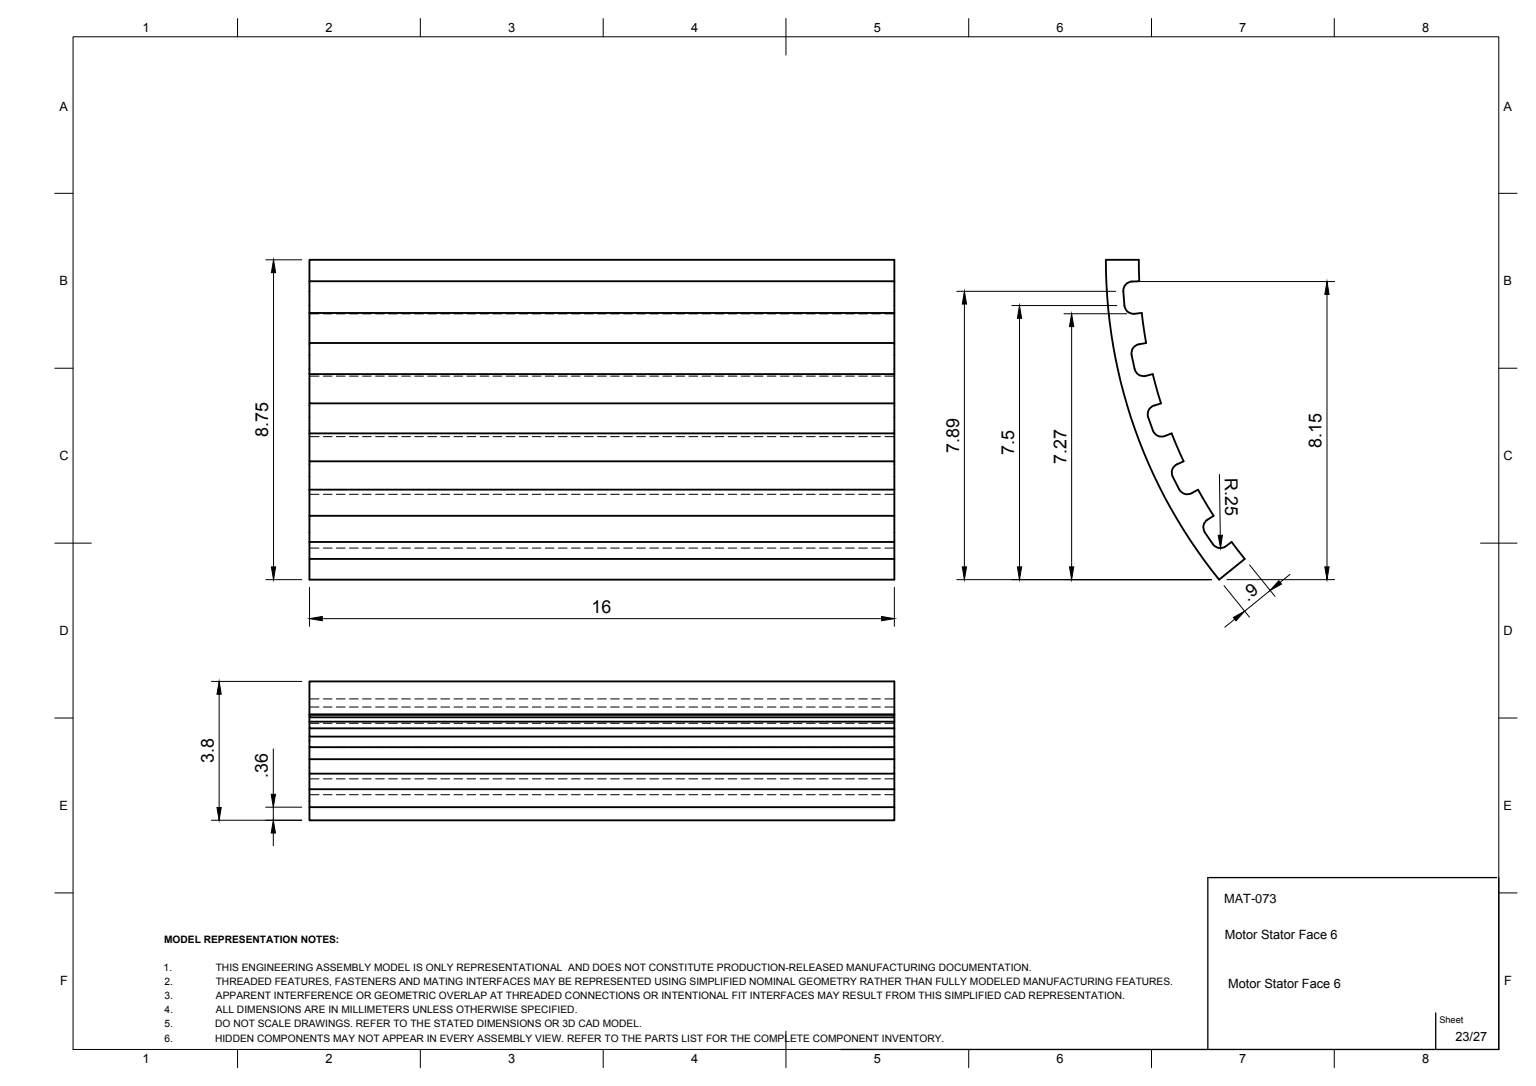
ISO-10303-21;
HEADER;
/* Generated by software containing ST-Developer
 * from STEP Tools, Inc. (www.steptools.com) 
 */

FILE_DESCRIPTION(
/* description */ ('CAx-IF Rec.Pracs.---Representation and Presentation of Product Manufa
cturing Information (PMI)---4.0---2014-10-13'),
/* implementation_level */ '2;1');

FILE_NAME(
/* name */ 'Motor Stator Face 6.step',
/* time_stamp */ '2026-10-24T18:52:33-07:00',
/* author */ (''),
/* organization */ (''),
/* preprocessor_version */ 'ST-DEVELOPER v20.2',
/* originating_system */ 'Autodesk Translation Framework v15.17.0.0',
/* authorisation */ '');

FILE_SCHEMA (('AP242_MANAGED_MODEL_BASED_3D_ENGINEERING_MIM_LF { 1 0 10303 442 2 1 4 }'));
ENDSEC;

DATA;
#10=MECHANICAL_DESIGN_GEOMETRIC_PRESENTATION_REPRESENTATION('',(#439),#34876);
#373=SHAPE_REPRESENTATION_RELATIONSHIP('SRR','None',#35010,#406);
#406=ADVANCED_BREP_SHAPE_REPRESENTATION('',(#472),#34868);
#439=STYLED_ITEM('',(#35160),#472);
#472=MANIFOLD_SOLID_BREP('Motor Stator Face 6',#19579);
#965=PLANE('',#21833);
#966=PLANE('',#21843);
#967=PLANE('',#21853);
#968=PLANE('',#21863);
#969=PLANE('',#21873);
#970=PLANE('',#21874);
#971=PLANE('',#21875);
#972=PLANE('',#21876);
#973=PLANE('',#21877);
#974=PLANE('',#21884);
#975=PLANE('',#21894);
#976=PLANE('',#21899);
#977=PLANE('',#21902);
#978=PLANE('',#21903);
#2305=LINE('',#33385,#3904);
#2306=LINE('',#33388,#3905);
#2307=LINE('',#33393,#3906);
#2308=LINE('',#33399,#3907);
#2309=LINE('',#33403,#3908);
#2310=LINE('',#33405,#3909);
#2311=LINE('',#33406,#3910);
#2312=LINE('',#33412,#3911);
#2313=LINE('',#33415,#3912);
#2314=LINE('',#33420,#3913);
#2315=LINE('',#33426,#3914);
#2316=LINE('',#33430,#3915);
#2317=LINE('',#33432,#3916);
#2318=LINE('',#33433,#3917);
#2319=LINE('',#33439,#3918);
#2320=LINE('',#33442,#3919);
#2321=LINE('',#33447,#3920);
#2322=LINE('',#33453,#3921);
#2323=LINE('',#33457,#3922);
#2324=LINE('',#33459,#3923);
#2325=LINE('',#33460,#3924);
#2326=LINE('',#33466,#3925);
#2327=LINE('',#33469,#3926);
#2328=LINE('',#33474,#3927);
#2329=LINE('',#33480,#3928);
#2330=LINE('',#33484,#3929);
#2331=LINE('',#33486,#3930);
#2332=LINE('',#33487,#3931);
#2333=LINE('',#33493,#3932);
#2334=LINE('',#33496,#3933);
#2335=LINE('',#33501,#3934);
#2336=LINE('',#33507,#3935);
#2337=LINE('',#33511,#3936);
#2338=LINE('',#33513,#3937);
#2339=LINE('',#33514,#3938);
#2340=LINE('',#33517,#3939);
#2341=LINE('',#33519,#3940);
#2342=LINE('',#33520,#3941);
#2343=LINE('',#33523,#3942);
#2344=LINE('',#33525,#3943);
#2345=LINE('',#33526,#3944);
#2346=LINE('',#33529,#3945);
#2347=LINE('',#33531,#3946);
#2348=LINE('',#33532,#3947);
#2349=LINE('',#33535,#3948);
#2350=LINE('',#33537,#3949);
#2351=LINE('',#33538,#3950);
#2352=LINE('',#33543,#3951);
#2353=LINE('',#33550,#3952);
#2354=LINE('',#33554,#3953);
#2355=LINE('',#33559,#3954);
#2356=LINE('',#33564,#3955);
#2357=LINE('',#33567,#3956);
#2358=LINE('',#33570,#3957);
#2359=LINE('',#33575,#3958);
#2360=LINE('',#33578,#3959);
#2361=LINE('',#33580,#3960);
#2362=LINE('',#33584,#3961);
#3904=VECTOR('',#27230,1.);
#3905=VECTOR('',#27233,1.);
#3906=VECTOR('',#27238,1.);
#3907=VECTOR('',#27245,1.);
#3908=VECTOR('',#27250,1.);
#3909=VECTOR('',#27251,1.);
#3910=VECTOR('',#27252,1.);
#3911=VECTOR('',#27257,1.);
#3912=VECTOR('',#27260,1.);
#3913=VECTOR('',#27265,1.);
#3914=VECTOR('',#27272,1.);
#3915=VECTOR('',#27277,1.);
#3916=VECTOR('',#27278,1.);
#3917=VECTOR('',#27279,1.);
#3918=VECTOR('',#27284,1.);
#3919=VECTOR('',#27287,1.);
#3920=VECTOR('',#27292,1.);
#3921=VECTOR('',#27299,1.);
#3922=VECTOR('',#27304,1.);
#3923=VECTOR('',#27305,1.);
#3924=VECTOR('',#27306,1.);
#3925=VECTOR('',#27311,1.);
#3926=VECTOR('',#27314,1.);
#3927=VECTOR('',#27319,1.);
#3928=VECTOR('',#27326,1.);
#3929=VECTOR('',#27331,1.);
#3930=VECTOR('',#27332,1.);
#3931=VECTOR('',#27333,1.);
#3932=VECTOR('',#27338,1.);
#3933=VECTOR('',#27341,1.);
#3934=VECTOR('',#27346,1.);
#3935=VECTOR('',#27353,1.);
#3936=VECTOR('',#27358,1.);
#3937=VECTOR('',#27359,1.);
#3938=VECTOR('',#27360,1.);
#3939=VECTOR('',#27363,1.);
#3940=VECTOR('',#27364,1.);
#3941=VECTOR('',#27365,1.);
#3942=VECTOR('',#27368,1.);
#3943=VECTOR('',#27369,1.);
#3944=VECTOR('',#27370,1.);
#3945=VECTOR('',#27373,1.);
#3946=VECTOR('',#27374,1.);
#3947=VECTOR('',#27375,1.);
#3948=VECTOR('',#27378,1.);
#3949=VECTOR('',#27379,1.);
#3950=VECTOR('',#27380,1.);
#3951=VECTOR('',#27385,1.);
#3952=VECTOR('',#27396,0.999999999999999);
#3953=VECTOR('',#27399,0.999999999999999);
#3954=VECTOR('',#27406,1.);
#3955=VECTOR('',#27413,1.);
#3956=VECTOR('',#27416,1.);
#3957=VECTOR('',#27421,1.);
#3958=VECTOR('',#27428,1.);
#3959=VECTOR('',#27431,1.);
#3960=VECTOR('',#27434,0.999999999999999);
#3961=VECTOR('',#27441,0.999999999999999);
#4720=CYLINDRICAL_SURFACE('',#21824,0.00025);
#4721=CYLINDRICAL_SURFACE('',#21827,0.01345);
#4722=CYLINDRICAL_SURFACE('',#21830,0.00025);
#4723=CYLINDRICAL_SURFACE('',#21834,0.00025);
#4724=CYLINDRICAL_SURFACE('',#21837,0.01345);
#4725=CYLINDRICAL_SURFACE('',#21840,0.00025);
#4726=CYLINDRICAL_SURFACE('',#21844,0.00025);
#4727=CYLINDRICAL_SURFACE('',#21847,0.01345);
#4728=CYLINDRICAL_SURFACE('',#21850,0.00025);
#4729=CYLINDRICAL_SURFACE('',#21854,0.00025);
#4730=CYLINDRICAL_SURFACE('',#21857,0.01345);
#4731=CYLINDRICAL_SURFACE('',#21860,0.00025);
#4732=CYLINDRICAL_SURFACE('',#21864,0.00025);
#4733=CYLINDRICAL_SURFACE('',#21867,0.01345);
#4734=CYLINDRICAL_SURFACE('',#21870,0.00025);
#4735=CYLINDRICAL_SURFACE('',#21878,0.013);
#4736=CYLINDRICAL_SURFACE('',#21881,0.013);
#4737=CYLINDRICAL_SURFACE('',#21890,0.013);
#4738=CYLINDRICAL_SURFACE('',#21892,0.013);
#4739=CYLINDRICAL_SURFACE('',#21895,0.013);
#4740=CYLINDRICAL_SURFACE('',#21897,0.0139);
#4741=CYLINDRICAL_SURFACE('',#21900,0.013);
#5627=FACE_OUTER_BOUND('',#6764,.T.);
#5628=FACE_OUTER_BOUND('',#6765,.T.);
#5629=FACE_OUTER_BOUND('',#6766,.T.);
#5630=FACE_OUTER_BOUND('',#6767,.T.);
#5631=FACE_OUTER_BOUND('',#6768,.T.);
#5632=FACE_OUTER_BOUND('',#6769,.T.);
#5633=FACE_OUTER_BOUND('',#6770,.T.);
#5634=FACE_OUTER_BOUND('',#6771,.T.);
#5635=FACE_OUTER_BOUND('',#6772,.T.);
#5636=FACE_OUTER_BOUND('',#6773,.T.);
#5637=FACE_OUTER_BOUND('',#6774,.T.);
#5638=FACE_OUTER_BOUND('',#6775,.T.);
#5639=FACE_OUTER_BOUND('',#6776,.T.);
#5640=FACE_OUTER_BOUND('',#6777,.T.);
#5641=FACE_OUTER_BOUND('',#6778,.T.);
#5642=FACE_OUTER_BOUND('',#6779,.T.);
#5643=FACE_OUTER_BOUND('',#6780,.T.);
#5644=FACE_OUTER_BOUND('',#6781,.T.);
#5645=FACE_OUTER_BOUND('',#6782,.T.);
#5646=FACE_OUTER_BOUND('',#6783,.T.);
#5647=FACE_OUTER_BOUND('',#6784,.T.);
#5648=FACE_OUTER_BOUND('',#6785,.T.);
#5649=FACE_OUTER_BOUND('',#6786,.T.);
#5650=FACE_OUTER_BOUND('',#6787,.T.);
#5651=FACE_OUTER_BOUND('',#6788,.T.);
#5652=FACE_OUTER_BOUND('',#6789,.T.);
#5653=FACE_OUTER_BOUND('',#6790,.T.);
#5654=FACE_OUTER_BOUND('',#6791,.T.);
#5655=FACE_OUTER_BOUND('',#6792,.T.);
#5656=FACE_OUTER_BOUND('',#6793,.T.);
#5657=FACE_OUTER_BOUND('',#6794,.T.);
#5658=FACE_OUTER_BOUND('',#6795,.T.);
#5659=FACE_OUTER_BOUND('',#6796,.T.);
#5660=FACE_OUTER_BOUND('',#6797,.T.);
#5661=FACE_OUTER_BOUND('',#6798,.T.);
#5662=FACE_OUTER_BOUND('',#6799,.T.);
#6764=EDGE_LOOP('',(#17318,#17319,#17320,#17321));
#6765=EDGE_LOOP('',(#17322,#17323,#17324,#17325));
#6766=EDGE_LOOP('',(#17326,#17327,#17328,#17329));
#6767=EDGE_LOOP('',(#17330,#17331,#17332,#17333));
#6768=EDGE_LOOP('',(#17334,#17335,#17336,#17337));
#6769=EDGE_LOOP('',(#17338,#17339,#17340,#17341));
#6770=EDGE_LOOP('',(#17342,#17343,#17344,#17345));
#6771=EDGE_LOOP('',(#17346,#17347,#17348,#17349));
#6772=EDGE_LOOP('',(#17350,#17351,#17352,#17353));
#6773=EDGE_LOOP('',(#17354,#17355,#17356,#17357));
#6774=EDGE_LOOP('',(#17358,#17359,#17360,#17361));
#6775=EDGE_LOOP('',(#17362,#17363,#17364,#17365));
#6776=EDGE_LOOP('',(#17366,#17367,#17368,#17369));
#6777=EDGE_LOOP('',(#17370,#17371,#17372,#17373));
#6778=EDGE_LOOP('',(#17374,#17375,#17376,#17377));
#6779=EDGE_LOOP('',(#17378,#17379,#17380,#17381));
#6780=EDGE_LOOP('',(#17382,#17383,#17384,#17385));
#6781=EDGE_LOOP('',(#17386,#17387,#17388,#17389));
#6782=EDGE_LOOP('',(#17390,#17391,#17392,#17393));
#6783=EDGE_LOOP('',(#17394,#17395,#17396,#17397));
#6784=EDGE_LOOP('',(#17398,#17399,#17400,#17401));
#6785=EDGE_LOOP('',(#17402,#17403,#17404,#17405));
#6786=EDGE_LOOP('',(#17406,#17407,#17408,#17409));
#6787=EDGE_LOOP('',(#17410,#17411,#17412,#17413));
#6788=EDGE_LOOP('',(#17414,#17415,#17416,#17417));
#6789=EDGE_LOOP('',(#17418,#17419,#17420,#17421));
#6790=EDGE_LOOP('',(#17422,#17423,#17424,#17425,#17426,#17427,#17428,#17429,
#17430,#17431,#17432,#17433,#17434,#17435,#17436,#17437,#17438,#17439,#17440,
#17441,#17442,#17443,#17444,#17445,#17446,#17447,#17448,#17449,#17450,#17451,
#17452,#17453,#17454,#17455));
#6791=EDGE_LOOP('',(#17456,#17457,#17458,#17459));
#6792=EDGE_LOOP('',(#17460,#17461,#17462,#17463));
#6793=EDGE_LOOP('',(#17464,#17465,#17466,#17467));
#6794=EDGE_LOOP('',(#17468,#17469,#17470,#17471));
#6795=EDGE_LOOP('',(#17472,#17473,#17474,#17475));
#6796=EDGE_LOOP('',(#17476,#17477,#17478,#17479));
#6797=EDGE_LOOP('',(#17480,#17481,#17482,#17483));
#6798=EDGE_LOOP('',(#17484,#17485,#17486,#17487));
#6799=EDGE_LOOP('',(#17488,#17489,#17490,#17491,#17492,#17493,#17494,#17495,
#17496,#17497,#17498,#17499,#17500,#17501,#17502,#17503,#17504,#17505,#17506,
#17507,#17508,#17509,#17510,#17511,#17512,#17513,#17514,#17515,#17516,#17517,
#17518,#17519,#17520,#17521));
#7893=CIRCLE('',#21825,0.000250000000013569);
#7894=CIRCLE('',#21826,0.000250000000013569);
#7895=CIRCLE('',#21828,0.0134500000000125);
#7896=CIRCLE('',#21829,0.0134500000000125);
#7897=CIRCLE('',#21831,0.000250000000013744);
#7898=CIRCLE('',#21832,0.000250000000013744);
#7899=CIRCLE('',#21835,0.000250000000013973);
#7900=CIRCLE('',#21836,0.000250000000013973);
#7901=CIRCLE('',#21838,0.0134500000000115);
#7902=CIRCLE('',#21839,0.0134500000000115);
#7903=CIRCLE('',#21841,0.000250000000014062);
#7904=CIRCLE('',#21842,0.000250000000014062);
#7905=CIRCLE('',#21845,0.000250000000014138);
#7906=CIRCLE('',#21846,0.000250000000014138);
#7907=CIRCLE('',#21848,0.0134500000000103);
#7908=CIRCLE('',#21849,0.0134500000000103);
#7909=CIRCLE('',#21851,0.000250000000014138);
#7910=CIRCLE('',#21852,0.000250000000014138);
#7911=CIRCLE('',#21855,0.000250000000014062);
#7912=CIRCLE('',#21856,0.000250000000014062);
#7913=CIRCLE('',#21858,0.0134500000000109);
#7914=CIRCLE('',#21859,0.0134500000000109);
#7915=CIRCLE('',#21861,0.000250000000013973);
#7916=CIRCLE('',#21862,0.000250000000013973);
#7917=CIRCLE('',#21865,0.000250000000013744);
#7918=CIRCLE('',#21866,0.000250000000013744);
#7919=CIRCLE('',#21868,0.013450000000012);
#7920=CIRCLE('',#21869,0.013450000000012);
#7921=CIRCLE('',#21871,0.000250000000013569);
#7922=CIRCLE('',#21872,0.000250000000013569);
#7923=CIRCLE('',#21879,0.0130000000000128);
#7924=CIRCLE('',#21880,0.0130000000000128);
#7925=CIRCLE('',#21882,0.0130000000000128);
#7926=CIRCLE('',#21883,0.0130000000000128);
#7927=CIRCLE('',#21885,0.0139000000000128);
#7928=CIRCLE('',#21886,0.0130000000000128);
#7929=CIRCLE('',#21887,0.0130000000000128);
#7930=CIRCLE('',#21888,0.0130000000000128);
#7931=CIRCLE('',#21889,0.0130000000000128);
#7932=CIRCLE('',#21891,0.0130000000000128);
#7933=CIRCLE('',#21893,0.0130000000000128);
#7934=CIRCLE('',#21896,0.0130000000000128);
#7935=CIRCLE('',#21898,0.0139000000000128);
#7936=CIRCLE('',#21901,0.0130000000000128);
#9569=VERTEX_POINT('',#33381);
#9570=VERTEX_POINT('',#33382);
#9571=VERTEX_POINT('',#33384);
#9572=VERTEX_POINT('',#33386);
#9573=VERTEX_POINT('',#33390);
#9574=VERTEX_POINT('',#33392);
#9575=VERTEX_POINT('',#33396);
#9576=VERTEX_POINT('',#33398);
#9577=VERTEX_POINT('',#33402);
#9578=VERTEX_POINT('',#33404);
#9579=VERTEX_POINT('',#33408);
#9580=VERTEX_POINT('',#33409);
#9581=VERTEX_POINT('',#33411);
#9582=VERTEX_POINT('',#33413);
#9583=VERTEX_POINT('',#33417);
#9584=VERTEX_POINT('',#33419);
#9585=VERTEX_POINT('',#33423);
#9586=VERTEX_POINT('',#33425);
#9587=VERTEX_POINT('',#33429);
#9588=VERTEX_POINT('',#33431);
#9589=VERTEX_POINT('',#33435);
#9590=VERTEX_POINT('',#33436);
#9591=VERTEX_POINT('',#33438);
#9592=VERTEX_POINT('',#33440);
#9593=VERTEX_POINT('',#33444);
#9594=VERTEX_POINT('',#33446);
#9595=VERTEX_POINT('',#33450);
#9596=VERTEX_POINT('',#33452);
#9597=VERTEX_POINT('',#33456);
#9598=VERTEX_POINT('',#33458);
#9599=VERTEX_POINT('',#33462);
#9600=VERTEX_POINT('',#33463);
#9601=VERTEX_POINT('',#33465);
#9602=VERTEX_POINT('',#33467);
#9603=VERTEX_POINT('',#33471);
#9604=VERTEX_POINT('',#33473);
#9605=VERTEX_POINT('',#33477);
#9606=VERTEX_POINT('',#33479);
#9607=VERTEX_POINT('',#33483);
#9608=VERTEX_POINT('',#33485);
#9609=VERTEX_POINT('',#33489);
#9610=VERTEX_POINT('',#33490);
#9611=VERTEX_POINT('',#33492);
#9612=VERTEX_POINT('',#33494);
#9613=VERTEX_POINT('',#33498);
#9614=VERTEX_POINT('',#33500);
#9615=VERTEX_POINT('',#33504);
#9616=VERTEX_POINT('',#33506);
#9617=VERTEX_POINT('',#33510);
#9618=VERTEX_POINT('',#33512);
#9619=VERTEX_POINT('',#33516);
#9620=VERTEX_POINT('',#33518);
#9621=VERTEX_POINT('',#33522);
#9622=VERTEX_POINT('',#33524);
#9623=VERTEX_POINT('',#33528);
#9624=VERTEX_POINT('',#33530);
#9625=VERTEX_POINT('',#33534);
#9626=VERTEX_POINT('',#33536);
#9627=VERTEX_POINT('',#33540);
#9628=VERTEX_POINT('',#33542);
#9629=VERTEX_POINT('',#33549);
#9630=VERTEX_POINT('',#33551);
#9631=VERTEX_POINT('',#33553);
#9632=VERTEX_POINT('',#33557);
#9633=VERTEX_POINT('',#33562);
#9634=VERTEX_POINT('',#33566);
#9635=VERTEX_POINT('',#33574);
#9636=VERTEX_POINT('',#33576);
#12217=EDGE_CURVE('',#9569,#9570,#7893,.T.);
#12218=EDGE_CURVE('',#9570,#9571,#2305,.T.);
#12219=EDGE_CURVE('',#9571,#9572,#7894,.T.);
#12220=EDGE_CURVE('',#9572,#9569,#2306,.T.);
#12221=EDGE_CURVE('',#9573,#9570,#7895,.T.);
#12222=EDGE_CURVE('',#9574,#9573,#2307,.T.);
#12223=EDGE_CURVE('',#9571,#9574,#7896,.T.);
#12224=EDGE_CURVE('',#9573,#9575,#7897,.T.);
#12225=EDGE_CURVE('',#9575,#9576,#2308,.T.);
#12226=EDGE_CURVE('',#9576,#9574,#7898,.T.);
#12227=EDGE_CURVE('',#9577,#9575,#2309,.T.);
#12228=EDGE_CURVE('',#9578,#9577,#2310,.T.);
#12229=EDGE_CURVE('',#9576,#9578,#2311,.T.);
#12230=EDGE_CURVE('',#9579,#9580,#7899,.T.);
#12231=EDGE_CURVE('',#9580,#9581,#2312,.T.);
#12232=EDGE_CURVE('',#9581,#9582,#7900,.T.);
#12233=EDGE_CURVE('',#9582,#9579,#2313,.T.);
#12234=EDGE_CURVE('',#9583,#9580,#7901,.T.);
#12235=EDGE_CURVE('',#9584,#9583,#2314,.T.);
#12236=EDGE_CURVE('',#9581,#9584,#7902,.T.);
#12237=EDGE_CURVE('',#9583,#9585,#7903,.T.);
#12238=EDGE_CURVE('',#9585,#9586,#2315,.T.);
#12239=EDGE_CURVE('',#9586,#9584,#7904,.T.);
#12240=EDGE_CURVE('',#9587,#9585,#2316,.T.);
#12241=EDGE_CURVE('',#9588,#9587,#2317,.T.);
#12242=EDGE_CURVE('',#9586,#9588,#2318,.T.);
#12243=EDGE_CURVE('',#9589,#9590,#7905,.T.);
#12244=EDGE_CURVE('',#9590,#9591,#2319,.T.);
#12245=EDGE_CURVE('',#9591,#9592,#7906,.T.);
#12246=EDGE_CURVE('',#9592,#9589,#2320,.T.);
#12247=EDGE_CURVE('',#9593,#9590,#7907,.T.);
#12248=EDGE_CURVE('',#9594,#9593,#2321,.T.);
#12249=EDGE_CURVE('',#9591,#9594,#7908,.T.);
#12250=EDGE_CURVE('',#9593,#9595,#7909,.T.);
#12251=EDGE_CURVE('',#9595,#9596,#2322,.T.);
#12252=EDGE_CURVE('',#9596,#9594,#7910,.T.);
#12253=EDGE_CURVE('',#9597,#9595,#2323,.T.);
#12254=EDGE_CURVE('',#9598,#9597,#2324,.T.);
#12255=EDGE_CURVE('',#9596,#9598,#2325,.T.);
#12256=EDGE_CURVE('',#9599,#9600,#7911,.T.);
#12257=EDGE_CURVE('',#9600,#9601,#2326,.T.);
#12258=EDGE_CURVE('',#9601,#9602,#7912,.T.);
#12259=EDGE_CURVE('',#9602,#9599,#2327,.T.);
#12260=EDGE_CURVE('',#9603,#9600,#7913,.T.);
#12261=EDGE_CURVE('',#9604,#9603,#2328,.T.);
#12262=EDGE_CURVE('',#9601,#9604,#7914,.T.);
#12263=EDGE_CURVE('',#9603,#9605,#7915,.T.);
#12264=EDGE_CURVE('',#9605,#9606,#2329,.T.);
#12265=EDGE_CURVE('',#9606,#9604,#7916,.T.);
#12266=EDGE_CURVE('',#9607,#9605,#2330,.T.);
#12267=EDGE_CURVE('',#9608,#9607,#2331,.T.);
#12268=EDGE_CURVE('',#9606,#9608,#2332,.T.);
#12269=EDGE_CURVE('',#9609,#9610,#7917,.T.);
#12270=EDGE_CURVE('',#9610,#9611,#2333,.T.);
#12271=EDGE_CURVE('',#9611,#9612,#7918,.T.);
#12272=EDGE_CURVE('',#9612,#9609,#2334,.T.);
#12273=EDGE_CURVE('',#9613,#9610,#7919,.T.);
#12274=EDGE_CURVE('',#9614,#9613,#2335,.T.);
#12275=EDGE_CURVE('',#9611,#9614,#7920,.T.);
#12276=EDGE_CURVE('',#9613,#9615,#7921,.T.);
#12277=EDGE_CURVE('',#9615,#9616,#2336,.T.);
#12278=EDGE_CURVE('',#9616,#9614,#7922,.T.);
#12279=EDGE_CURVE('',#9617,#9615,#2337,.T.);
#12280=EDGE_CURVE('',#9618,#9617,#2338,.T.);
#12281=EDGE_CURVE('',#9616,#9618,#2339,.T.);
#12282=EDGE_CURVE('',#9619,#9612,#2340,.T.);
#12283=EDGE_CURVE('',#9620,#9619,#2341,.T.);
#12284=EDGE_CURVE('',#9609,#9620,#2342,.T.);
#12285=EDGE_CURVE('',#9621,#9602,#2343,.T.);
#12286=EDGE_CURVE('',#9622,#9621,#2344,.T.);
#12287=EDGE_CURVE('',#9599,#9622,#2345,.T.);
#12288=EDGE_CURVE('',#9623,#9582,#2346,.T.);
#12289=EDGE_CURVE('',#9624,#9623,#2347,.T.);
#12290=EDGE_CURVE('',#9579,#9624,#2348,.T.);
#12291=EDGE_CURVE('',#9625,#9572,#2349,.T.);
#12292=EDGE_CURVE('',#9626,#9625,#2350,.T.);
#12293=EDGE_CURVE('',#9569,#9626,#2351,.T.);
#12294=EDGE_CURVE('',#9627,#9617,#7923,.T.);
#12295=EDGE_CURVE('',#9628,#9627,#2352,.T.);
#12296=EDGE_CURVE('',#9618,#9628,#7924,.T.);
#12297=EDGE_CURVE('',#9598,#9621,#7925,.T.);
#12298=EDGE_CURVE('',#9622,#9597,#7926,.T.);
#12299=EDGE_CURVE('',#9628,#9629,#2353,.T.);
#12300=EDGE_CURVE('',#9629,#9630,#7927,.T.);
#12301=EDGE_CURVE('',#9630,#9631,#2354,.T.);
#12302=EDGE_CURVE('',#9631,#9625,#7928,.T.);
#12303=EDGE_CURVE('',#9578,#9623,#7929,.T.);
#12304=EDGE_CURVE('',#9588,#9632,#7930,.T.);
#12305=EDGE_CURVE('',#9632,#9592,#2355,.T.);
#12306=EDGE_CURVE('',#9608,#9619,#7931,.T.);
#12307=EDGE_CURVE('',#9633,#9587,#7932,.T.);
#12308=EDGE_CURVE('',#9633,#9632,#2356,.T.);
#12309=EDGE_CURVE('',#9631,#9634,#2357,.T.);
#12310=EDGE_CURVE('',#9626,#9634,#7933,.T.);
#12311=EDGE_CURVE('',#9589,#9633,#2358,.T.);
#12312=EDGE_CURVE('',#9620,#9607,#7934,.T.);
#12313=EDGE_CURVE('',#9635,#9629,#2359,.T.);
#12314=EDGE_CURVE('',#9636,#9635,#7935,.T.);
#12315=EDGE_CURVE('',#9630,#9636,#2360,.T.);
#12316=EDGE_CURVE('',#9634,#9636,#2361,.T.);
#12317=EDGE_CURVE('',#9624,#9577,#7936,.T.);
#12318=EDGE_CURVE('',#9635,#9627,#2362,.T.);
#17318=ORIENTED_EDGE('',*,*,#12217,.T.);
#17319=ORIENTED_EDGE('',*,*,#12218,.T.);
#17320=ORIENTED_EDGE('',*,*,#12219,.T.);
#17321=ORIENTED_EDGE('',*,*,#12220,.T.);
#17322=ORIENTED_EDGE('',*,*,#12218,.F.);
#17323=ORIENTED_EDGE('',*,*,#12221,.F.);
#17324=ORIENTED_EDGE('',*,*,#12222,.F.);
#17325=ORIENTED_EDGE('',*,*,#12223,.F.);
#17326=ORIENTED_EDGE('',*,*,#12224,.T.);
#17327=ORIENTED_EDGE('',*,*,#12225,.T.);
#17328=ORIENTED_EDGE('',*,*,#12226,.T.);
#17329=ORIENTED_EDGE('',*,*,#12222,.T.);
#17330=ORIENTED_EDGE('',*,*,#12225,.F.);
#17331=ORIENTED_EDGE('',*,*,#12227,.F.);
#17332=ORIENTED_EDGE('',*,*,#12228,.F.);
#17333=ORIENTED_EDGE('',*,*,#12229,.F.);
#17334=ORIENTED_EDGE('',*,*,#12230,.T.);
#17335=ORIENTED_EDGE('',*,*,#12231,.T.);
#17336=ORIENTED_EDGE('',*,*,#12232,.T.);
#17337=ORIENTED_EDGE('',*,*,#12233,.T.);
#17338=ORIENTED_EDGE('',*,*,#12231,.F.);
#17339=ORIENTED_EDGE('',*,*,#12234,.F.);
#17340=ORIENTED_EDGE('',*,*,#12235,.F.);
#17341=ORIENTED_EDGE('',*,*,#12236,.F.);
#17342=ORIENTED_EDGE('',*,*,#12237,.T.);
#17343=ORIENTED_EDGE('',*,*,#12238,.T.);
#17344=ORIENTED_EDGE('',*,*,#12239,.T.);
#17345=ORIENTED_EDGE('',*,*,#12235,.T.);
#17346=ORIENTED_EDGE('',*,*,#12238,.F.);
#17347=ORIENTED_EDGE('',*,*,#12240,.F.);
#17348=ORIENTED_EDGE('',*,*,#12241,.F.);
#17349=ORIENTED_EDGE('',*,*,#12242,.F.);
#17350=ORIENTED_EDGE('',*,*,#12243,.T.);
#17351=ORIENTED_EDGE('',*,*,#12244,.T.);
#17352=ORIENTED_EDGE('',*,*,#12245,.T.);
#17353=ORIENTED_EDGE('',*,*,#12246,.T.);
#17354=ORIENTED_EDGE('',*,*,#12244,.F.);
#17355=ORIENTED_EDGE('',*,*,#12247,.F.);
#17356=ORIENTED_EDGE('',*,*,#12248,.F.);
#17357=ORIENTED_EDGE('',*,*,#12249,.F.);
#17358=ORIENTED_EDGE('',*,*,#12250,.T.);
#17359=ORIENTED_EDGE('',*,*,#12251,.T.);
#17360=ORIENTED_EDGE('',*,*,#12252,.T.);
#17361=ORIENTED_EDGE('',*,*,#12248,.T.);
#17362=ORIENTED_EDGE('',*,*,#12251,.F.);
#17363=ORIENTED_EDGE('',*,*,#12253,.F.);
#17364=ORIENTED_EDGE('',*,*,#12254,.F.);
#17365=ORIENTED_EDGE('',*,*,#12255,.F.);
#17366=ORIENTED_EDGE('',*,*,#12256,.T.);
#17367=ORIENTED_EDGE('',*,*,#12257,.T.);
#17368=ORIENTED_EDGE('',*,*,#12258,.T.);
#17369=ORIENTED_EDGE('',*,*,#12259,.T.);
#17370=ORIENTED_EDGE('',*,*,#12257,.F.);
#17371=ORIENTED_EDGE('',*,*,#12260,.F.);
#17372=ORIENTED_EDGE('',*,*,#12261,.F.);
#17373=ORIENTED_EDGE('',*,*,#12262,.F.);
#17374=ORIENTED_EDGE('',*,*,#12263,.T.);
#17375=ORIENTED_EDGE('',*,*,#12264,.T.);
#17376=ORIENTED_EDGE('',*,*,#12265,.T.);
#17377=ORIENTED_EDGE('',*,*,#12261,.T.);
#17378=ORIENTED_EDGE('',*,*,#12264,.F.);
#17379=ORIENTED_EDGE('',*,*,#12266,.F.);
#17380=ORIENTED_EDGE('',*,*,#12267,.F.);
#17381=ORIENTED_EDGE('',*,*,#12268,.F.);
#17382=ORIENTED_EDGE('',*,*,#12269,.T.);
#17383=ORIENTED_EDGE('',*,*,#12270,.T.);
#17384=ORIENTED_EDGE('',*,*,#12271,.T.);
#17385=ORIENTED_EDGE('',*,*,#12272,.T.);
#17386=ORIENTED_EDGE('',*,*,#12270,.F.);
#17387=ORIENTED_EDGE('',*,*,#12273,.F.);
#17388=ORIENTED_EDGE('',*,*,#12274,.F.);
#17389=ORIENTED_EDGE('',*,*,#12275,.F.);
#17390=ORIENTED_EDGE('',*,*,#12276,.T.);
#17391=ORIENTED_EDGE('',*,*,#12277,.T.);
#17392=ORIENTED_EDGE('',*,*,#12278,.T.);
#17393=ORIENTED_EDGE('',*,*,#12274,.T.);
#17394=ORIENTED_EDGE('',*,*,#12277,.F.);
#17395=ORIENTED_EDGE('',*,*,#12279,.F.);
#17396=ORIENTED_EDGE('',*,*,#12280,.F.);
#17397=ORIENTED_EDGE('',*,*,#12281,.F.);
#17398=ORIENTED_EDGE('',*,*,#12272,.F.);
#17399=ORIENTED_EDGE('',*,*,#12282,.F.);
#17400=ORIENTED_EDGE('',*,*,#12283,.F.);
#17401=ORIENTED_EDGE('',*,*,#12284,.F.);
#17402=ORIENTED_EDGE('',*,*,#12259,.F.);
#17403=ORIENTED_EDGE('',*,*,#12285,.F.);
#17404=ORIENTED_EDGE('',*,*,#12286,.F.);
#17405=ORIENTED_EDGE('',*,*,#12287,.F.);
#17406=ORIENTED_EDGE('',*,*,#12233,.F.);
#17407=ORIENTED_EDGE('',*,*,#12288,.F.);
#17408=ORIENTED_EDGE('',*,*,#12289,.F.);
#17409=ORIENTED_EDGE('',*,*,#12290,.F.);
#17410=ORIENTED_EDGE('',*,*,#12220,.F.);
#17411=ORIENTED_EDGE('',*,*,#12291,.F.);
#17412=ORIENTED_EDGE('',*,*,#12292,.F.);
#17413=ORIENTED_EDGE('',*,*,#12293,.F.);
#17414=ORIENTED_EDGE('',*,*,#12280,.T.);
#17415=ORIENTED_EDGE('',*,*,#12294,.F.);
#17416=ORIENTED_EDGE('',*,*,#12295,.F.);
#17417=ORIENTED_EDGE('',*,*,#12296,.F.);
#17418=ORIENTED_EDGE('',*,*,#12286,.T.);
#17419=ORIENTED_EDGE('',*,*,#12297,.F.);
#17420=ORIENTED_EDGE('',*,*,#12254,.T.);
#17421=ORIENTED_EDGE('',*,*,#12298,.F.);
#17422=ORIENTED_EDGE('',*,*,#12282,.T.);
#17423=ORIENTED_EDGE('',*,*,#12271,.F.);
#17424=ORIENTED_EDGE('',*,*,#12275,.T.);
#17425=ORIENTED_EDGE('',*,*,#12278,.F.);
#17426=ORIENTED_EDGE('',*,*,#12281,.T.);
#17427=ORIENTED_EDGE('',*,*,#12296,.T.);
#17428=ORIENTED_EDGE('',*,*,#12299,.T.);
#17429=ORIENTED_EDGE('',*,*,#12300,.T.);
#17430=ORIENTED_EDGE('',*,*,#12301,.T.);
#17431=ORIENTED_EDGE('',*,*,#12302,.T.);
#17432=ORIENTED_EDGE('',*,*,#12291,.T.);
#17433=ORIENTED_EDGE('',*,*,#12219,.F.);
#17434=ORIENTED_EDGE('',*,*,#12223,.T.);
#17435=ORIENTED_EDGE('',*,*,#12226,.F.);
#17436=ORIENTED_EDGE('',*,*,#12229,.T.);
#17437=ORIENTED_EDGE('',*,*,#12303,.T.);
#17438=ORIENTED_EDGE('',*,*,#12288,.T.);
#17439=ORIENTED_EDGE('',*,*,#12232,.F.);
#17440=ORIENTED_EDGE('',*,*,#12236,.T.);
#17441=ORIENTED_EDGE('',*,*,#12239,.F.);
#17442=ORIENTED_EDGE('',*,*,#12242,.T.);
#17443=ORIENTED_EDGE('',*,*,#12304,.T.);
#17444=ORIENTED_EDGE('',*,*,#12305,.T.);
#17445=ORIENTED_EDGE('',*,*,#12245,.F.);
#17446=ORIENTED_EDGE('',*,*,#12249,.T.);
#17447=ORIENTED_EDGE('',*,*,#12252,.F.);
#17448=ORIENTED_EDGE('',*,*,#12255,.T.);
#17449=ORIENTED_EDGE('',*,*,#12297,.T.);
#17450=ORIENTED_EDGE('',*,*,#12285,.T.);
#17451=ORIENTED_EDGE('',*,*,#12258,.F.);
#17452=ORIENTED_EDGE('',*,*,#12262,.T.);
#17453=ORIENTED_EDGE('',*,*,#12265,.F.);
#17454=ORIENTED_EDGE('',*,*,#12268,.T.);
#17455=ORIENTED_EDGE('',*,*,#12306,.T.);
#17456=ORIENTED_EDGE('',*,*,#12241,.T.);
#17457=ORIENTED_EDGE('',*,*,#12307,.F.);
#17458=ORIENTED_EDGE('',*,*,#12308,.T.);
#17459=ORIENTED_EDGE('',*,*,#12304,.F.);
#17460=ORIENTED_EDGE('',*,*,#12292,.T.);
#17461=ORIENTED_EDGE('',*,*,#12302,.F.);
#17462=ORIENTED_EDGE('',*,*,#12309,.T.);
#17463=ORIENTED_EDGE('',*,*,#12310,.F.);
#17464=ORIENTED_EDGE('',*,*,#12246,.F.);
#17465=ORIENTED_EDGE('',*,*,#12305,.F.);
#17466=ORIENTED_EDGE('',*,*,#12308,.F.);
#17467=ORIENTED_EDGE('',*,*,#12311,.F.);
#17468=ORIENTED_EDGE('',*,*,#12283,.T.);
#17469=ORIENTED_EDGE('',*,*,#12306,.F.);
#17470=ORIENTED_EDGE('',*,*,#12267,.T.);
#17471=ORIENTED_EDGE('',*,*,#12312,.F.);
#17472=ORIENTED_EDGE('',*,*,#12313,.F.);
#17473=ORIENTED_EDGE('',*,*,#12314,.F.);
#17474=ORIENTED_EDGE('',*,*,#12315,.F.);
#17475=ORIENTED_EDGE('',*,*,#12300,.F.);
#17476=ORIENTED_EDGE('',*,*,#12315,.T.);
#17477=ORIENTED_EDGE('',*,*,#12316,.F.);
#17478=ORIENTED_EDGE('',*,*,#12309,.F.);
#17479=ORIENTED_EDGE('',*,*,#12301,.F.);
#17480=ORIENTED_EDGE('',*,*,#12289,.T.);
#17481=ORIENTED_EDGE('',*,*,#12303,.F.);
#17482=ORIENTED_EDGE('',*,*,#12228,.T.);
#17483=ORIENTED_EDGE('',*,*,#12317,.F.);
#17484=ORIENTED_EDGE('',*,*,#12295,.T.);
#17485=ORIENTED_EDGE('',*,*,#12318,.F.);
#17486=ORIENTED_EDGE('',*,*,#12313,.T.);
#17487=ORIENTED_EDGE('',*,*,#12299,.F.);
#17488=ORIENTED_EDGE('',*,*,#12284,.T.);
#17489=ORIENTED_EDGE('',*,*,#12312,.T.);
#17490=ORIENTED_EDGE('',*,*,#12266,.T.);
#17491=ORIENTED_EDGE('',*,*,#12263,.F.);
#17492=ORIENTED_EDGE('',*,*,#12260,.T.);
#17493=ORIENTED_EDGE('',*,*,#12256,.F.);
#17494=ORIENTED_EDGE('',*,*,#12287,.T.);
#17495=ORIENTED_EDGE('',*,*,#12298,.T.);
#17496=ORIENTED_EDGE('',*,*,#12253,.T.);
#17497=ORIENTED_EDGE('',*,*,#12250,.F.);
#17498=ORIENTED_EDGE('',*,*,#12247,.T.);
#17499=ORIENTED_EDGE('',*,*,#12243,.F.);
#17500=ORIENTED_EDGE('',*,*,#12311,.T.);
#17501=ORIENTED_EDGE('',*,*,#12307,.T.);
#17502=ORIENTED_EDGE('',*,*,#12240,.T.);
#17503=ORIENTED_EDGE('',*,*,#12237,.F.);
#17504=ORIENTED_EDGE('',*,*,#12234,.T.);
#17505=ORIENTED_EDGE('',*,*,#12230,.F.);
#17506=ORIENTED_EDGE('',*,*,#12290,.T.);
#17507=ORIENTED_EDGE('',*,*,#12317,.T.);
#17508=ORIENTED_EDGE('',*,*,#12227,.T.);
#17509=ORIENTED_EDGE('',*,*,#12224,.F.);
#17510=ORIENTED_EDGE('',*,*,#12221,.T.);
#17511=ORIENTED_EDGE('',*,*,#12217,.F.);
#17512=ORIENTED_EDGE('',*,*,#12293,.T.);
#17513=ORIENTED_EDGE('',*,*,#12310,.T.);
#17514=ORIENTED_EDGE('',*,*,#12316,.T.);
#17515=ORIENTED_EDGE('',*,*,#12314,.T.);
#17516=ORIENTED_EDGE('',*,*,#12318,.T.);
#17517=ORIENTED_EDGE('',*,*,#12294,.T.);
#17518=ORIENTED_EDGE('',*,*,#12279,.T.);
#17519=ORIENTED_EDGE('',*,*,#12276,.F.);
#17520=ORIENTED_EDGE('',*,*,#12273,.T.);
#17521=ORIENTED_EDGE('',*,*,#12269,.F.);
#19343=ADVANCED_FACE('',(#5627),#4720,.F.);
#19344=ADVANCED_FACE('',(#5628),#4721,.F.);
#19345=ADVANCED_FACE('',(#5629),#4722,.F.);
#19346=ADVANCED_FACE('',(#5630),#965,.F.);
#19347=ADVANCED_FACE('',(#5631),#4723,.F.);
#19348=ADVANCED_FACE('',(#5632),#4724,.F.);
#19349=ADVANCED_FACE('',(#5633),#4725,.F.);
#19350=ADVANCED_FACE('',(#5634),#966,.F.);
#19351=ADVANCED_FACE('',(#5635),#4726,.F.);
#19352=ADVANCED_FACE('',(#5636),#4727,.F.);
#19353=ADVANCED_FACE('',(#5637),#4728,.F.);
#19354=ADVANCED_FACE('',(#5638),#967,.F.);
#19355=ADVANCED_FACE('',(#5639),#4729,.F.);
#19356=ADVANCED_FACE('',(#5640),#4730,.F.);
#19357=ADVANCED_FACE('',(#5641),#4731,.F.);
#19358=ADVANCED_FACE('',(#5642),#968,.F.);
#19359=ADVANCED_FACE('',(#5643),#4732,.F.);
#19360=ADVANCED_FACE('',(#5644),#4733,.F.);
#19361=ADVANCED_FACE('',(#5645),#4734,.F.);
#19362=ADVANCED_FACE('',(#5646),#969,.F.);
#19363=ADVANCED_FACE('',(#5647),#970,.F.);
#19364=ADVANCED_FACE('',(#5648),#971,.F.);
#19365=ADVANCED_FACE('',(#5649),#972,.F.);
#19366=ADVANCED_FACE('',(#5650),#973,.F.);
#19367=ADVANCED_FACE('',(#5651),#4735,.F.);
#19368=ADVANCED_FACE('',(#5652),#4736,.F.);
#19369=ADVANCED_FACE('',(#5653),#974,.F.);
#19370=ADVANCED_FACE('',(#5654),#4737,.F.);
#19371=ADVANCED_FACE('',(#5655),#4738,.F.);
#19372=ADVANCED_FACE('',(#5656),#975,.F.);
#19373=ADVANCED_FACE('',(#5657),#4739,.F.);
#19374=ADVANCED_FACE('',(#5658),#4740,.T.);
#19375=ADVANCED_FACE('',(#5659),#976,.T.);
#19376=ADVANCED_FACE('',(#5660),#4741,.F.);
#19377=ADVANCED_FACE('',(#5661),#977,.T.);
#19378=ADVANCED_FACE('',(#5662),#978,.T.);
#19579=CLOSED_SHELL('',(#19343,#19344,#19345,#19346,#19347,#19348,#19349,
#19350,#19351,#19352,#19353,#19354,#19355,#19356,#19357,#19358,#19359,#19360,
#19361,#19362,#19363,#19364,#19365,#19366,#19367,#19368,#19369,#19370,#19371,
#19372,#19373,#19374,#19375,#19376,#19377,#19378));
#21823=AXIS2_PLACEMENT_3D('',#33379,#27224,#27225);
#21824=AXIS2_PLACEMENT_3D('',#33380,#27226,#27227);
#21825=AXIS2_PLACEMENT_3D('',#33383,#27228,#27229);
#21826=AXIS2_PLACEMENT_3D('',#33387,#27231,#27232);
#21827=AXIS2_PLACEMENT_3D('',#33389,#27234,#27235);
#21828=AXIS2_PLACEMENT_3D('',#33391,#27236,#27237);
#21829=AXIS2_PLACEMENT_3D('',#33394,#27239,#27240);
#21830=AXIS2_PLACEMENT_3D('',#33395,#27241,#27242);
#21831=AXIS2_PLACEMENT_3D('',#33397,#27243,#27244);
#21832=AXIS2_PLACEMENT_3D('',#33400,#27246,#27247);
#21833=AXIS2_PLACEMENT_3D('',#33401,#27248,#27249);
#21834=AXIS2_PLACEMENT_3D('',#33407,#27253,#27254);
#21835=AXIS2_PLACEMENT_3D('',#33410,#27255,#27256);
#21836=AXIS2_PLACEMENT_3D('',#33414,#27258,#27259);
#21837=AXIS2_PLACEMENT_3D('',#33416,#27261,#27262);
#21838=AXIS2_PLACEMENT_3D('',#33418,#27263,#27264);
#21839=AXIS2_PLACEMENT_3D('',#33421,#27266,#27267);
#21840=AXIS2_PLACEMENT_3D('',#33422,#27268,#27269);
#21841=AXIS2_PLACEMENT_3D('',#33424,#27270,#27271);
#21842=AXIS2_PLACEMENT_3D('',#33427,#27273,#27274);
#21843=AXIS2_PLACEMENT_3D('',#33428,#27275,#27276);
#21844=AXIS2_PLACEMENT_3D('',#33434,#27280,#27281);
#21845=AXIS2_PLACEMENT_3D('',#33437,#27282,#27283);
#21846=AXIS2_PLACEMENT_3D('',#33441,#27285,#27286);
#21847=AXIS2_PLACEMENT_3D('',#33443,#27288,#27289);
#21848=AXIS2_PLACEMENT_3D('',#33445,#27290,#27291);
#21849=AXIS2_PLACEMENT_3D('',#33448,#27293,#27294);
#21850=AXIS2_PLACEMENT_3D('',#33449,#27295,#27296);
#21851=AXIS2_PLACEMENT_3D('',#33451,#27297,#27298);
#21852=AXIS2_PLACEMENT_3D('',#33454,#27300,#27301);
#21853=AXIS2_PLACEMENT_3D('',#33455,#27302,#27303);
#21854=AXIS2_PLACEMENT_3D('',#33461,#27307,#27308);
#21855=AXIS2_PLACEMENT_3D('',#33464,#27309,#27310);
#21856=AXIS2_PLACEMENT_3D('',#33468,#27312,#27313);
#21857=AXIS2_PLACEMENT_3D('',#33470,#27315,#27316);
#21858=AXIS2_PLACEMENT_3D('',#33472,#27317,#27318);
#21859=AXIS2_PLACEMENT_3D('',#33475,#27320,#27321);
#21860=AXIS2_PLACEMENT_3D('',#33476,#27322,#27323);
#21861=AXIS2_PLACEMENT_3D('',#33478,#27324,#27325);
#21862=AXIS2_PLACEMENT_3D('',#33481,#27327,#27328);
#21863=AXIS2_PLACEMENT_3D('',#33482,#27329,#27330);
#21864=AXIS2_PLACEMENT_3D('',#33488,#27334,#27335);
#21865=AXIS2_PLACEMENT_3D('',#33491,#27336,#27337);
#21866=AXIS2_PLACEMENT_3D('',#33495,#27339,#27340);
#21867=AXIS2_PLACEMENT_3D('',#33497,#27342,#27343);
#21868=AXIS2_PLACEMENT_3D('',#33499,#27344,#27345);
#21869=AXIS2_PLACEMENT_3D('',#33502,#27347,#27348);
#21870=AXIS2_PLACEMENT_3D('',#33503,#27349,#27350);
#21871=AXIS2_PLACEMENT_3D('',#33505,#27351,#27352);
#21872=AXIS2_PLACEMENT_3D('',#33508,#27354,#27355);
#21873=AXIS2_PLACEMENT_3D('',#33509,#27356,#27357);
#21874=AXIS2_PLACEMENT_3D('',#33515,#27361,#27362);
#21875=AXIS2_PLACEMENT_3D('',#33521,#27366,#27367);
#21876=AXIS2_PLACEMENT_3D('',#33527,#27371,#27372);
#21877=AXIS2_PLACEMENT_3D('',#33533,#27376,#27377);
#21878=AXIS2_PLACEMENT_3D('',#33539,#27381,#27382);
#21879=AXIS2_PLACEMENT_3D('',#33541,#27383,#27384);
#21880=AXIS2_PLACEMENT_3D('',#33544,#27386,#27387);
#21881=AXIS2_PLACEMENT_3D('',#33545,#27388,#27389);
#21882=AXIS2_PLACEMENT_3D('',#33546,#27390,#27391);
#21883=AXIS2_PLACEMENT_3D('',#33547,#27392,#27393);
#21884=AXIS2_PLACEMENT_3D('',#33548,#27394,#27395);
#21885=AXIS2_PLACEMENT_3D('',#33552,#27397,#27398);
#21886=AXIS2_PLACEMENT_3D('',#33555,#27400,#27401);
#21887=AXIS2_PLACEMENT_3D('',#33556,#27402,#27403);
#21888=AXIS2_PLACEMENT_3D('',#33558,#27404,#27405);
#21889=AXIS2_PLACEMENT_3D('',#33560,#27407,#27408);
#21890=AXIS2_PLACEMENT_3D('',#33561,#27409,#27410);
#21891=AXIS2_PLACEMENT_3D('',#33563,#27411,#27412);
#21892=AXIS2_PLACEMENT_3D('',#33565,#27414,#27415);
#21893=AXIS2_PLACEMENT_3D('',#33568,#27417,#27418);
#21894=AXIS2_PLACEMENT_3D('',#33569,#27419,#27420);
#21895=AXIS2_PLACEMENT_3D('',#33571,#27422,#27423);
#21896=AXIS2_PLACEMENT_3D('',#33572,#27424,#27425);
#21897=AXIS2_PLACEMENT_3D('',#33573,#27426,#27427);
#21898=AXIS2_PLACEMENT_3D('',#33577,#27429,#27430);
#21899=AXIS2_PLACEMENT_3D('',#33579,#27432,#27433);
#21900=AXIS2_PLACEMENT_3D('',#33581,#27435,#27436);
#21901=AXIS2_PLACEMENT_3D('',#33582,#27437,#27438);
#21902=AXIS2_PLACEMENT_3D('',#33583,#27439,#27440);
#21903=AXIS2_PLACEMENT_3D('',#33585,#27442,#27443);
#27224=DIRECTION('axis',(0.,0.,1.));
#27225=DIRECTION('refdir',(1.,0.,0.));
#27226=DIRECTION('center_axis',(0.,-1.,0.));
#27227=DIRECTION('ref_axis',(-0.877771605587211,0.,0.479079334165908));
#27228=DIRECTION('center_axis',(0.,1.,0.));
#27229=DIRECTION('ref_axis',(-0.877771605579571,0.,0.479079334179906));
#27230=DIRECTION('',(0.,-1.,0.));
#27231=DIRECTION('center_axis',(0.,-1.,0.));
#27232=DIRECTION('ref_axis',(-0.877771605579571,0.,0.479079334179906));
#27233=DIRECTION('',(0.,1.,0.));
#27234=DIRECTION('center_axis',(0.,-1.,0.));
#27235=DIRECTION('ref_axis',(-0.290991366091359,0.,0.956725679001188));
#27236=DIRECTION('center_axis',(0.,-1.,0.));
#27237=DIRECTION('ref_axis',(-0.290991366091832,0.,0.956725679001044));
#27238=DIRECTION('',(0.,1.,0.));
#27239=DIRECTION('center_axis',(0.,1.,0.));
#27240=DIRECTION('ref_axis',(-0.290991366091832,0.,0.956725679001044));
#27241=DIRECTION('center_axis',(0.,-1.,0.));
#27242=DIRECTION('ref_axis',(0.520632842076226,0.,0.853780676609416));
#27243=DIRECTION('center_axis',(0.,1.,0.));
#27244=DIRECTION('ref_axis',(0.520632842087603,0.,0.853780676602478));
#27245=DIRECTION('',(0.,-1.,0.));
#27246=DIRECTION('center_axis',(0.,-1.,0.));
#27247=DIRECTION('ref_axis',(0.520632842087603,0.,0.853780676602478));
#27248=DIRECTION('center_axis',(0.974044425513625,0.,0.22635692418354));
#27249=DIRECTION('ref_axis',(0.,-1.,0.));
#27250=DIRECTION('',(-0.226356924184268,0.,0.974044425513455));
#27251=DIRECTION('',(0.,1.,0.));
#27252=DIRECTION('',(0.226356924184268,0.,-0.974044425513455));
#27253=DIRECTION('center_axis',(0.,-1.,0.));
#27254=DIRECTION('ref_axis',(-0.80772974655928,0.,0.589552929365364));
#27255=DIRECTION('center_axis',(0.,1.,0.));
#27256=DIRECTION('ref_axis',(-0.807729746554134,0.,0.589552929372413));
#27257=DIRECTION('',(0.,-1.,0.));
#27258=DIRECTION('center_axis',(0.,-1.,0.));
#27259=DIRECTION('ref_axis',(-0.807729746554134,0.,0.589552929372413));
#27260=DIRECTION('',(0.,1.,0.));
#27261=DIRECTION('center_axis',(0.,-1.,0.));
#27262=DIRECTION('ref_axis',(-0.163624134736254,0.,0.986522753174914));
#27263=DIRECTION('center_axis',(0.,-1.,0.));
#27264=DIRECTION('ref_axis',(-0.163624134736857,0.,0.986522753174814));
#27265=DIRECTION('',(0.,1.,0.));
#27266=DIRECTION('center_axis',(0.,1.,0.));
#27267=DIRECTION('ref_axis',(-0.163624134736857,0.,0.986522753174814));
#27268=DIRECTION('center_axis',(0.,-1.,0.));
#27269=DIRECTION('ref_axis',(0.627619496647803,0.,0.778520242143747));
#27270=DIRECTION('center_axis',(0.,1.,0.));
#27271=DIRECTION('ref_axis',(0.627619496652502,0.,0.778520242139959));
#27272=DIRECTION('',(0.,-1.,0.));
#27273=DIRECTION('center_axis',(0.,-1.,0.));
#27274=DIRECTION('ref_axis',(0.627619496652502,0.,0.778520242139959));
#27275=DIRECTION('center_axis',(0.995256847821609,0.,0.0972820994026908));
#27276=DIRECTION('ref_axis',(0.,-1.,0.));
#27277=DIRECTION('',(-0.0972820994035846,0.,0.995256847821521));
#27278=DIRECTION('',(0.,1.,0.));
#27279=DIRECTION('',(0.0972820994035846,0.,-0.995256847821521));
#27280=DIRECTION('center_axis',(0.,-1.,0.));
#27281=DIRECTION('ref_axis',(-0.723867407622732,0.,0.689939110488415));
#27282=DIRECTION('center_axis',(0.,1.,0.));
#27283=DIRECTION('ref_axis',(-0.723867407621795,0.,0.689939110489398));
#27284=DIRECTION('',(0.,-1.,0.));
#27285=DIRECTION('center_axis',(0.,-1.,0.));
#27286=DIRECTION('ref_axis',(-0.723867407621795,0.,0.689939110489398));
#27287=DIRECTION('',(0.,1.,0.));
#27288=DIRECTION('center_axis',(0.,-1.,0.));
#27289=DIRECTION('ref_axis',(-0.033457249070632,0.,0.999440149526036));
#27290=DIRECTION('center_axis',(0.,-1.,0.));
#27291=DIRECTION('ref_axis',(-0.0334572490713498,0.,0.999440149526012));
#27292=DIRECTION('',(0.,1.,0.));
#27293=DIRECTION('center_axis',(0.,1.,0.));
#27294=DIRECTION('ref_axis',(-0.0334572490713498,0.,0.999440149526012));
#27295=DIRECTION('center_axis',(0.,-1.,0.));
#27296=DIRECTION('ref_axis',(0.723867407622732,0.,0.689939110488415));
#27297=DIRECTION('center_axis',(0.,1.,0.));
#27298=DIRECTION('ref_axis',(0.723867407621795,0.,0.689939110489398));
#27299=DIRECTION('',(0.,-1.,0.));
#27300=DIRECTION('center_axis',(0.,-1.,0.));
#27301=DIRECTION('ref_axis',(0.723867407621795,0.,0.689939110489398));
#27302=DIRECTION('center_axis',(0.999440149526036,0.,-0.0334572490706319));
#27303=DIRECTION('ref_axis',(0.,-1.,0.));
#27304=DIRECTION('',(0.0334572490715974,0.,0.999440149526004));
#27305=DIRECTION('',(0.,1.,0.));
#27306=DIRECTION('',(-0.0334572490715974,0.,-0.999440149526004));
#27307=DIRECTION('center_axis',(0.,-1.,0.));
#27308=DIRECTION('ref_axis',(-0.627619496647803,0.,0.778520242143747));
#27309=DIRECTION('center_axis',(0.,1.,0.));
#27310=DIRECTION('ref_axis',(-0.627619496652502,0.,0.778520242139959));
#27311=DIRECTION('',(0.,-1.,0.));
#27312=DIRECTION('center_axis',(0.,-1.,0.));
#27313=DIRECTION('ref_axis',(-0.627619496652502,0.,0.778520242139959));
#27314=DIRECTION('',(0.,1.,0.));
#27315=DIRECTION('center_axis',(0.,-1.,0.));
#27316=DIRECTION('ref_axis',(0.0972820994026908,0.,0.995256847821609));
#27317=DIRECTION('center_axis',(0.,-1.,0.));
#27318=DIRECTION('ref_axis',(0.0972820994033552,0.,0.995256847821544));
#27319=DIRECTION('',(0.,1.,0.));
#27320=DIRECTION('center_axis',(0.,1.,0.));
#27321=DIRECTION('ref_axis',(0.0972820994033552,0.,0.995256847821544));
#27322=DIRECTION('center_axis',(0.,-1.,0.));
#27323=DIRECTION('ref_axis',(0.807729746559285,0.,0.589552929365357));
#27324=DIRECTION('center_axis',(0.,1.,0.));
#27325=DIRECTION('ref_axis',(0.80772974655414,0.,0.589552929372406));
#27326=DIRECTION('',(0.,-1.,0.));
#27327=DIRECTION('center_axis',(0.,-1.,0.));
#27328=DIRECTION('ref_axis',(0.80772974655414,0.,0.589552929372406));
#27329=DIRECTION('center_axis',(0.986522753174914,0.,-0.163624134736254));
#27330=DIRECTION('ref_axis',(0.,-1.,0.));
#27331=DIRECTION('',(0.163624134737066,0.,0.986522753174779));
#27332=DIRECTION('',(0.,1.,0.));
#27333=DIRECTION('',(-0.163624134737066,0.,-0.986522753174779));
#27334=DIRECTION('center_axis',(0.,-1.,0.));
#27335=DIRECTION('ref_axis',(-0.520632842076221,0.,0.853780676609419));
#27336=DIRECTION('center_axis',(0.,1.,0.));
#27337=DIRECTION('ref_axis',(-0.520632842087598,0.,0.853780676602481));
#27338=DIRECTION('',(0.,-1.,0.));
#27339=DIRECTION('center_axis',(0.,-1.,0.));
#27340=DIRECTION('ref_axis',(-0.520632842087598,0.,0.853780676602481));
#27341=DIRECTION('',(0.,1.,0.));
#27342=DIRECTION('center_axis',(0.,-1.,0.));
#27343=DIRECTION('ref_axis',(0.22635692418354,0.,0.974044425513625));
#27344=DIRECTION('center_axis',(0.,-1.,0.));
#27345=DIRECTION('ref_axis',(0.226356924184081,0.,0.974044425513499));
#27346=DIRECTION('',(0.,1.,0.));
#27347=DIRECTION('center_axis',(0.,1.,0.));
#27348=DIRECTION('ref_axis',(0.226356924184081,0.,0.974044425513499));
#27349=DIRECTION('center_axis',(0.,-1.,0.));
#27350=DIRECTION('ref_axis',(0.877771605587212,0.,0.479079334165907));
#27351=DIRECTION('center_axis',(0.,1.,0.));
#27352=DIRECTION('ref_axis',(0.877771605579571,0.,0.479079334179906));
#27353=DIRECTION('',(0.,-1.,0.));
#27354=DIRECTION('center_axis',(0.,-1.,0.));
#27355=DIRECTION('ref_axis',(0.877771605579571,0.,0.479079334179906));
#27356=DIRECTION('center_axis',(0.956725679001188,0.,-0.290991366091359));
#27357=DIRECTION('ref_axis',(0.,-1.,0.));
#27358=DIRECTION('',(0.290991366091996,0.,0.956725679000994));
#27359=DIRECTION('',(0.,1.,0.));
#27360=DIRECTION('',(-0.290991366091996,0.,-0.956725679000994));
#27361=DIRECTION('center_axis',(-0.974044425513625,0.,0.22635692418354));
#27362=DIRECTION('ref_axis',(0.,1.,0.));
#27363=DIRECTION('',(0.226356924184268,0.,0.974044425513455));
#27364=DIRECTION('',(0.,-1.,0.));
#27365=DIRECTION('',(-0.226356924184268,0.,-0.974044425513455));
#27366=DIRECTION('center_axis',(-0.995256847821609,0.,0.0972820994026909));
#27367=DIRECTION('ref_axis',(0.,1.,0.));
#27368=DIRECTION('',(0.0972820994035846,0.,0.995256847821521));
#27369=DIRECTION('',(0.,-1.,0.));
#27370=DIRECTION('',(-0.0972820994035846,0.,-0.995256847821521));
#27371=DIRECTION('center_axis',(-0.986522753174914,0.,-0.163624134736254));
#27372=DIRECTION('ref_axis',(-0.163624134736254,0.,0.986522753174914));
#27373=DIRECTION('',(-0.163624134737066,0.,0.986522753174779));
#27374=DIRECTION('',(0.,-1.,0.));
#27375=DIRECTION('',(0.163624134737066,0.,-0.986522753174779));
#27376=DIRECTION('center_axis',(-0.956725679001188,0.,-0.290991366091359));
#27377=DIRECTION('ref_axis',(-0.290991366091359,0.,0.956725679001188));
#27378=DIRECTION('',(-0.290991366091996,0.,0.956725679000994));
#27379=DIRECTION('',(0.,-1.,0.));
#27380=DIRECTION('',(0.290991366091996,0.,-0.956725679000994));
#27381=DIRECTION('center_axis',(0.,1.,0.));
#27382=DIRECTION('ref_axis',(0.333806859233771,0.,-0.942641491092178));
#27383=DIRECTION('center_axis',(0.,-1.,0.));
#27384=DIRECTION('ref_axis',(0.333806859234212,0.,-0.942641491092022));
#27385=DIRECTION('',(0.,1.,0.));
#27386=DIRECTION('center_axis',(0.,1.,0.));
#27387=DIRECTION('ref_axis',(0.333806859234212,0.,-0.942641491092022));
#27388=DIRECTION('center_axis',(0.,1.,0.));
#27389=DIRECTION('ref_axis',(0.333806859233771,0.,-0.942641491092178));
#27390=DIRECTION('center_axis',(0.,1.,0.));
#27391=DIRECTION('ref_axis',(0.333806859234212,0.,-0.942641491092022));
#27392=DIRECTION('center_axis',(0.,-1.,0.));
#27393=DIRECTION('ref_axis',(0.333806859234212,0.,-0.942641491092022));
#27394=DIRECTION('center_axis',(0.,1.,0.));
#27395=DIRECTION('ref_axis',(1.,0.,0.));
#27396=DIRECTION('',(0.333806859234347,0.,0.942641491091974));
#27397=DIRECTION('center_axis',(0.,-1.,0.));
#27398=DIRECTION('ref_axis',(-0.333806859234184,0.,0.942641491092032));
#27399=DIRECTION('',(0.333806859234347,0.,-0.942641491091974));
#27400=DIRECTION('center_axis',(0.,1.,0.));
#27401=DIRECTION('ref_axis',(0.333806859234212,0.,-0.942641491092022));
#27402=DIRECTION('center_axis',(0.,1.,0.));
#27403=DIRECTION('ref_axis',(0.333806859234212,0.,-0.942641491092022));
#27404=DIRECTION('center_axis',(0.,1.,0.));
#27405=DIRECTION('ref_axis',(0.333806859234212,0.,-0.942641491092022));
#27406=DIRECTION('',(-0.0334572490715974,0.,0.999440149526004));
#27407=DIRECTION('center_axis',(0.,1.,0.));
#27408=DIRECTION('ref_axis',(0.333806859234212,0.,-0.942641491092022));
#27409=DIRECTION('center_axis',(0.,1.,0.));
#27410=DIRECTION('ref_axis',(0.333806859233771,0.,-0.942641491092178));
#27411=DIRECTION('center_axis',(0.,-1.,0.));
#27412=DIRECTION('ref_axis',(0.333806859234212,0.,-0.942641491092022));
#27413=DIRECTION('',(0.,-1.,0.));
#27414=DIRECTION('center_axis',(0.,1.,0.));
#27415=DIRECTION('ref_axis',(0.333806859233771,0.,-0.942641491092178));
#27416=DIRECTION('',(0.,1.,0.));
#27417=DIRECTION('center_axis',(0.,-1.,0.));
#27418=DIRECTION('ref_axis',(0.333806859234212,0.,-0.942641491092022));
#27419=DIRECTION('center_axis',(-0.999440149526036,0.,-0.0334572490706319));
#27420=DIRECTION('ref_axis',(-0.0334572490706319,0.,0.999440149526036));
#27421=DIRECTION('',(0.0334572490715974,0.,-0.999440149526004));
#27422=DIRECTION('center_axis',(0.,1.,0.));
#27423=DIRECTION('ref_axis',(0.333806859233771,0.,-0.942641491092178));
#27424=DIRECTION('center_axis',(0.,-1.,0.));
#27425=DIRECTION('ref_axis',(0.333806859234212,0.,-0.942641491092022));
#27426=DIRECTION('center_axis',(0.,1.,0.));
#27427=DIRECTION('ref_axis',(-0.333806859233771,0.,0.942641491092178));
#27428=DIRECTION('',(0.,-1.,0.));
#27429=DIRECTION('center_axis',(0.,1.,0.));
#27430=DIRECTION('ref_axis',(-0.333806859234184,0.,0.942641491092032));
#27431=DIRECTION('',(0.,1.,0.));
#27432=DIRECTION('center_axis',(-0.942641491092178,0.,-0.333806859233773));
#27433=DIRECTION('ref_axis',(-0.333806859233773,0.,0.942641491092178));
#27434=DIRECTION('',(-0.333806859234347,0.,0.942641491091974));
#27435=DIRECTION('center_axis',(0.,1.,0.));
#27436=DIRECTION('ref_axis',(0.333806859233771,0.,-0.942641491092178));
#27437=DIRECTION('center_axis',(0.,-1.,0.));
#27438=DIRECTION('ref_axis',(0.333806859234212,0.,-0.942641491092022));
#27439=DIRECTION('center_axis',(0.942641491092178,0.,-0.333806859233773));
#27440=DIRECTION('ref_axis',(0.,-1.,0.));
#27441=DIRECTION('',(-0.333806859234347,0.,-0.942641491091974));
#27442=DIRECTION('center_axis',(0.,1.,0.));
#27443=DIRECTION('ref_axis',(1.,0.,0.));
#33379=CARTESIAN_POINT('',(0.,0.,0.));
#33380=CARTESIAN_POINT('Origin',(-0.00360121565085295,-0.008,0.0126992616256242));
#33381=CARTESIAN_POINT('',(-0.00384039707060325,-0.008,0.0126265137841014));
#33382=CARTESIAN_POINT('',(-0.00366942049272517,-0.008,0.0129397779442914));
#33383=CARTESIAN_POINT('Origin',(-0.00360121565086296,-0.00799999999999,
0.0126992616256342));
#33384=CARTESIAN_POINT('',(-0.00366942049272517,-0.024,0.0129397779442914));
#33385=CARTESIAN_POINT('',(-0.00366942049273517,-0.00799999999999,0.0129397779443014));
#33386=CARTESIAN_POINT('',(-0.00384039707060325,-0.024,0.0126265137841014));
#33387=CARTESIAN_POINT('Origin',(-0.00360121565086296,-0.02400000000001,
0.0126992616256342));
#33388=CARTESIAN_POINT('',(-0.00384039707061325,-0.00799999999999,0.0126265137841114));
#33389=CARTESIAN_POINT('Origin',(-4.44089209850063E-17,-0.008,6.72997231505748E-33));
#33390=CARTESIAN_POINT('',(-0.00329207760827854,-0.008,0.0130408866654485));
#33391=CARTESIAN_POINT('Origin',(-4.44089209850063E-17,-0.00799999999999,
6.72997231505748E-33));
#33392=CARTESIAN_POINT('',(-0.00329207760827854,-0.024,0.0130408866654485));
#33393=CARTESIAN_POINT('',(-0.00329207760828854,-0.00799999999999,0.0130408866654585));
#33394=CARTESIAN_POINT('Origin',(-4.44089209850063E-17,-0.02400000000001,
6.72997231505748E-33));
#33395=CARTESIAN_POINT('Origin',(-0.00323088657466742,-0.008,0.0127984910025219));
#33396=CARTESIAN_POINT('',(-0.00298737546828901,-0.008,0.0128550802335678));
#33397=CARTESIAN_POINT('Origin',(-0.00323088657467743,-0.00799999999999,
0.0127984910025319));
#33398=CARTESIAN_POINT('',(-0.00298737546828901,-0.024,0.0128550802335678));
#33399=CARTESIAN_POINT('',(-0.00298737546829902,-0.00799999999999,0.0128550802335778));
#33400=CARTESIAN_POINT('Origin',(-0.00323088657467743,-0.02400000000001,
0.0127984910025319));
#33401=CARTESIAN_POINT('Origin',(-0.00294264001438606,-0.008,0.0126625775316771));
#33402=CARTESIAN_POINT('',(-0.00294264001438606,-0.008,0.0126625775316771));
#33403=CARTESIAN_POINT('',(-0.00291295831081416,-0.00799999999999,0.0125348531511851));
#33404=CARTESIAN_POINT('',(-0.00294264001438606,-0.024,0.0126625775316771));
#33405=CARTESIAN_POINT('',(-0.00294264001439606,-0.016,0.0126625775316871));
#33406=CARTESIAN_POINT('',(-0.00291295831081416,-0.02400000000001,0.0125348531511851));
#33407=CARTESIAN_POINT('Origin',(-0.00191282048773815,-0.008,0.0130606706482359));
#33408=CARTESIAN_POINT('',(-0.00215945117603188,-0.008,0.0130197646145518));
#33409=CARTESIAN_POINT('',(-0.00194904814849077,-0.008,0.0133080318347555));
#33410=CARTESIAN_POINT('Origin',(-0.00191282048774815,-0.00799999999999,
0.0130606706482459));
#33411=CARTESIAN_POINT('',(-0.00194904814849077,-0.024,0.0133080318347555));
#33412=CARTESIAN_POINT('',(-0.00194904814850077,-0.00799999999999,0.0133080318347655));
#33413=CARTESIAN_POINT('',(-0.00215945117603188,-0.024,0.0130197646145518));
#33414=CARTESIAN_POINT('Origin',(-0.00191282048774815,-0.02400000000001,
0.0130606706482459));
#33415=CARTESIAN_POINT('',(-0.00215945117604188,-0.00799999999999,0.0130197646145618));
#33416=CARTESIAN_POINT('Origin',(-4.44089209850063E-17,-0.008,6.72997231505748E-33));
#33417=CARTESIAN_POINT('',(-0.00156173614835732,-0.008,0.0133590224269186));
#33418=CARTESIAN_POINT('Origin',(-4.44089209850063E-17,-0.00799999999999,
6.72997231505748E-33));
#33419=CARTESIAN_POINT('',(-0.00156173614835732,-0.024,0.0133590224269186));
#33420=CARTESIAN_POINT('',(-0.00156173614836731,-0.00799999999999,0.0133590224269286));
#33421=CARTESIAN_POINT('Origin',(-4.44089209850063E-17,-0.02400000000001,
6.72997231505748E-33));
#33422=CARTESIAN_POINT('Origin',(-0.00153270759541388,-0.008,0.0131107134598755));
#33423=CARTESIAN_POINT('',(-0.00128389338345847,-0.008,0.0131350339847262));
#33424=CARTESIAN_POINT('Origin',(-0.00153270759542387,-0.00799999999999,
0.0131107134598855));
#33425=CARTESIAN_POINT('',(-0.00128389338345847,-0.024,0.0131350339847262));
#33426=CARTESIAN_POINT('',(-0.00128389338346847,-0.00799999999999,0.0131350339847362));
#33427=CARTESIAN_POINT('Origin',(-0.00153270759542387,-0.02400000000001,
0.0131107134598855));
#33428=CARTESIAN_POINT('Origin',(-0.00126466729223502,-0.008,0.0129383390216809));
#33429=CARTESIAN_POINT('',(-0.00126466729223502,-0.008,0.0129383390216809));
#33430=CARTESIAN_POINT('',(-0.00126540384839645,-0.00799999999999,0.0129458744527519));
#33431=CARTESIAN_POINT('',(-0.00126466729223502,-0.024,0.0129383390216809));
#33432=CARTESIAN_POINT('',(-0.00126466729224502,-0.016,0.0129383390216909));
#33433=CARTESIAN_POINT('',(-0.00126540384839645,-0.02400000000001,0.0129458744527519));
#33434=CARTESIAN_POINT('Origin',(-0.000191696435744125,-0.008,0.0131986079749541));
#33435=CARTESIAN_POINT('',(-0.000441556473125634,-0.008,0.0131902436626865));
#33436=CARTESIAN_POINT('',(-0.00019532705005746,-0.008,0.0134485816108434));
#33437=CARTESIAN_POINT('Origin',(-0.000191696435754125,-0.00799999999999,
0.0131986079749641));
#33438=CARTESIAN_POINT('',(-0.00019532705005746,-0.024,0.0134485816108434));
#33439=CARTESIAN_POINT('',(-0.00019532705006746,-0.00799999999999,0.0134485816108534));
#33440=CARTESIAN_POINT('',(-0.000441556473125634,-0.024,0.0131902436626865));
#33441=CARTESIAN_POINT('Origin',(-0.000191696435754125,-0.02400000000001,
0.0131986079749641));
#33442=CARTESIAN_POINT('',(-0.000441556473135633,-0.00799999999999,0.0131902436626965));
#33443=CARTESIAN_POINT('Origin',(-4.44089209850063E-17,-0.008,6.72997231505748E-33));
#33444=CARTESIAN_POINT('',(0.000195327050057369,-0.008,0.0134485816108434));
#33445=CARTESIAN_POINT('Origin',(-4.44089209850063E-17,-0.00799999999999,
6.72997231505748E-33));
#33446=CARTESIAN_POINT('',(0.000195327050057369,-0.024,0.0134485816108434));
#33447=CARTESIAN_POINT('',(0.000195327050067369,-0.00799999999999,0.0134485816108534));
#33448=CARTESIAN_POINT('Origin',(-4.44089209850063E-17,-0.02400000000001,
6.72997231505748E-33));
#33449=CARTESIAN_POINT('Origin',(0.000191696435744034,-0.008,0.0131986079749541));
#33450=CARTESIAN_POINT('',(0.000441556473125544,-0.008,0.0131902436626865));
#33451=CARTESIAN_POINT('Origin',(0.000191696435754034,-0.00799999999999,
0.0131986079749641));
#33452=CARTESIAN_POINT('',(0.000441556473125544,-0.024,0.0131902436626865));
#33453=CARTESIAN_POINT('',(0.000441556473135544,-0.00799999999999,0.0131902436626965));
#33454=CARTESIAN_POINT('Origin',(0.000191696435754034,-0.02400000000001,
0.0131986079749641));
#33455=CARTESIAN_POINT('Origin',(0.000434944237918172,-0.008,0.0129927219438385));
#33456=CARTESIAN_POINT('',(0.000434944237918172,-0.008,0.0129927219438385));
#33457=CARTESIAN_POINT('',(0.000436112706128989,-0.00799999999999,0.0130276266077339));
#33458=CARTESIAN_POINT('',(0.000434944237918172,-0.024,0.0129927219438385));
#33459=CARTESIAN_POINT('',(0.000434944237928171,-0.016,0.0129927219438485));
#33460=CARTESIAN_POINT('',(0.000436112706128989,-0.02400000000001,0.0130276266077339));
#33461=CARTESIAN_POINT('Origin',(0.00153270759541378,-0.008,0.0131107134598755));
#33462=CARTESIAN_POINT('',(0.00128389338345839,-0.008,0.0131350339847262));
#33463=CARTESIAN_POINT('',(0.00156173614835723,-0.008,0.0133590224269186));
#33464=CARTESIAN_POINT('Origin',(0.00153270759542378,-0.00799999999999,
0.0131107134598855));
#33465=CARTESIAN_POINT('',(0.00156173614835723,-0.024,0.0133590224269186));
#33466=CARTESIAN_POINT('',(0.00156173614836722,-0.00799999999999,0.0133590224269286));
#33467=CARTESIAN_POINT('',(0.00128389338345839,-0.024,0.0131350339847262));
#33468=CARTESIAN_POINT('Origin',(0.00153270759542378,-0.02400000000001,
0.0131107134598855));
#33469=CARTESIAN_POINT('',(0.00128389338346839,-0.00799999999999,0.0131350339847362));
#33470=CARTESIAN_POINT('Origin',(-4.44089209850063E-17,-0.008,6.72997231505748E-33));
#33471=CARTESIAN_POINT('',(0.00194904814849068,-0.008,0.0133080318347555));
#33472=CARTESIAN_POINT('Origin',(-4.44089209850063E-17,-0.00799999999999,
6.72997231505748E-33));
#33473=CARTESIAN_POINT('',(0.00194904814849068,-0.024,0.0133080318347555));
#33474=CARTESIAN_POINT('',(0.00194904814850068,-0.00799999999999,0.0133080318347655));
#33475=CARTESIAN_POINT('Origin',(-4.44089209850063E-17,-0.02400000000001,
6.72997231505748E-33));
#33476=CARTESIAN_POINT('Origin',(0.00191282048773806,-0.008,0.0130606706482359));
#33477=CARTESIAN_POINT('',(0.00215945117603179,-0.008,0.0130197646145518));
#33478=CARTESIAN_POINT('Origin',(0.00191282048774806,-0.00799999999999,
0.0130606706482459));
#33479=CARTESIAN_POINT('',(0.00215945117603179,-0.024,0.0130197646145518));
#33480=CARTESIAN_POINT('',(0.0021594511760418,-0.00799999999999,0.0130197646145618));
#33481=CARTESIAN_POINT('Origin',(0.00191282048774806,-0.02400000000001,
0.0130606706482459));
#33482=CARTESIAN_POINT('Origin',(0.00212711375157126,-0.008,0.0128247957912739));
#33483=CARTESIAN_POINT('',(0.00212711375157126,-0.008,0.0128247957912739));
#33484=CARTESIAN_POINT('',(0.00211900825769009,-0.00799999999999,0.0127759261415696));
#33485=CARTESIAN_POINT('',(0.00212711375157126,-0.024,0.0128247957912739));
#33486=CARTESIAN_POINT('',(0.00212711375158127,-0.016,0.0128247957912839));
#33487=CARTESIAN_POINT('',(0.00211900825769009,-0.02400000000001,0.0127759261415696));
#33488=CARTESIAN_POINT('Origin',(0.00323088657466734,-0.008,0.0127984910025219));
#33489=CARTESIAN_POINT('',(0.00298737546828893,-0.008,0.0128550802335678));
#33490=CARTESIAN_POINT('',(0.00329207760827845,-0.008,0.0130408866654485));
#33491=CARTESIAN_POINT('Origin',(0.00323088657467733,-0.00799999999999,
0.0127984910025319));
#33492=CARTESIAN_POINT('',(0.00329207760827845,-0.024,0.0130408866654485));
#33493=CARTESIAN_POINT('',(0.00329207760828845,-0.00799999999999,0.0130408866654585));
#33494=CARTESIAN_POINT('',(0.00298737546828893,-0.024,0.0128550802335678));
#33495=CARTESIAN_POINT('Origin',(0.00323088657467733,-0.02400000000001,
0.0127984910025319));
#33496=CARTESIAN_POINT('',(0.00298737546829892,-0.00799999999999,0.0128550802335778));
#33497=CARTESIAN_POINT('Origin',(-4.44089209850063E-17,-0.008,6.72997231505748E-33));
#33498=CARTESIAN_POINT('',(0.00366942049272508,-0.008,0.0129397779442914));
#33499=CARTESIAN_POINT('Origin',(-4.44089209850063E-17,-0.00799999999999,
6.72997231505748E-33));
#33500=CARTESIAN_POINT('',(0.00366942049272508,-0.024,0.0129397779442914));
#33501=CARTESIAN_POINT('',(0.00366942049273508,-0.00799999999999,0.0129397779443014));
#33502=CARTESIAN_POINT('Origin',(-4.44089209850063E-17,-0.02400000000001,
6.72997231505748E-33));
#33503=CARTESIAN_POINT('Origin',(0.00360121565085287,-0.008,0.0126992616256242));
#33504=CARTESIAN_POINT('',(0.00384039707060316,-0.008,0.0126265137841014));
#33505=CARTESIAN_POINT('Origin',(0.00360121565086286,-0.00799999999999,
0.0126992616256342));
#33506=CARTESIAN_POINT('',(0.00384039707060316,-0.024,0.0126265137841014));
#33507=CARTESIAN_POINT('',(0.00384039707061316,-0.00799999999999,0.0126265137841114));
#33508=CARTESIAN_POINT('Origin',(0.00360121565086286,-0.02400000000001,
0.0126992616256342));
#33509=CARTESIAN_POINT('Origin',(0.00378288775918762,-0.008,0.0124374338270155));
#33510=CARTESIAN_POINT('',(0.00378288775918762,-0.008,0.0124374338270155));
#33511=CARTESIAN_POINT('',(0.00371177878877259,-0.00799999999999,0.0122036407116943));
#33512=CARTESIAN_POINT('',(0.00378288775918762,-0.024,0.0124374338270155));
#33513=CARTESIAN_POINT('',(0.00378288775919761,-0.016,0.0124374338270255));
#33514=CARTESIAN_POINT('',(0.00371177878877259,-0.02400000000001,0.0122036407116943));
#33515=CARTESIAN_POINT('Origin',(0.00304450063026857,-0.008,0.0131008975231583));
#33516=CARTESIAN_POINT('',(0.00294264001438597,-0.024,0.0126625775316771));
#33517=CARTESIAN_POINT('',(0.00296388861875537,-0.02400000000001,0.0127540131469256));
#33518=CARTESIAN_POINT('',(0.00294264001438597,-0.008,0.0126625775316771));
#33519=CARTESIAN_POINT('',(0.00294264001439597,-0.016,0.0126625775316871));
#33520=CARTESIAN_POINT('',(0.00296388861875537,-0.00799999999999,0.0127540131469256));
#33521=CARTESIAN_POINT('Origin',(0.00130844423696615,-0.008,0.0133862046032006));
#33522=CARTESIAN_POINT('',(0.00126466729223494,-0.024,0.0129383390216809));
#33523=CARTESIAN_POINT('',(0.00128729232076197,-0.02400000000001,0.0131698072435117));
#33524=CARTESIAN_POINT('',(0.00126466729223494,-0.008,0.0129383390216809));
#33525=CARTESIAN_POINT('',(0.00126466729224494,-0.016,0.0129383390216909));
#33526=CARTESIAN_POINT('',(0.00128729232076197,-0.00799999999999,0.0131698072435117));
#33527=CARTESIAN_POINT('Origin',(-0.00220074461220267,-0.008,0.0132687310302026));
#33528=CARTESIAN_POINT('',(-0.00212711375157135,-0.024,0.0128247957912739));
#33529=CARTESIAN_POINT('',(-0.00215582368800584,-0.02400000000001,0.0129978937610339));
#33530=CARTESIAN_POINT('',(-0.00212711375157135,-0.008,0.0128247957912739));
#33531=CARTESIAN_POINT('',(-0.00212711375158134,-0.016,0.0128247957912839));
#33532=CARTESIAN_POINT('',(-0.00215582368800584,-0.00799999999999,0.0129978937610339));
#33533=CARTESIAN_POINT('Origin',(-0.00391383387392881,-0.008,0.012867960382566));
#33534=CARTESIAN_POINT('',(-0.0037828877591877,-0.024,0.0124374338270155));
#33535=CARTESIAN_POINT('',(-0.00377725184614322,-0.02400000000001,0.0124189039894696));
#33536=CARTESIAN_POINT('',(-0.0037828877591877,-0.008,0.0124374338270155));
#33537=CARTESIAN_POINT('',(-0.00378288775919771,-0.016,0.0124374338270255));
#33538=CARTESIAN_POINT('',(-0.00377725184614322,-0.00799999999999,0.0124189039894696));
#33539=CARTESIAN_POINT('Origin',(-4.44089209850063E-17,-0.016,6.72997231505748E-33));
#33540=CARTESIAN_POINT('',(0.00433948917003898,-0.008,0.0122543393841983));
#33541=CARTESIAN_POINT('Origin',(-4.44089209850063E-17,-0.00799999999999,
6.72997231505748E-33));
#33542=CARTESIAN_POINT('',(0.00433948917003898,-0.024,0.0122543393841983));
#33543=CARTESIAN_POINT('',(0.00433948917004898,-0.016,0.0122543393842083));
#33544=CARTESIAN_POINT('Origin',(-4.44089209850063E-17,-0.02400000000001,
6.72997231505748E-33));
#33545=CARTESIAN_POINT('Origin',(-4.44089209850063E-17,-0.016,6.72997231505748E-33));
#33546=CARTESIAN_POINT('Origin',(-4.44089209850063E-17,-0.02400000000001,
6.72997231505748E-33));
#33547=CARTESIAN_POINT('Origin',(-4.44089209850063E-17,-0.00799999999999,
6.72997231505748E-33));
#33548=CARTESIAN_POINT('Origin',(-4.57966997657877E-17,-0.024,0.0130771696920992));
#33549=CARTESIAN_POINT('',(0.00463991534334938,-0.024,0.0131027167261813));
#33550=CARTESIAN_POINT('',(0.00463991534335938,-0.02400000000001,0.0131027167261913));
#33551=CARTESIAN_POINT('',(-0.00463991534334946,-0.024,0.0131027167261813));
#33552=CARTESIAN_POINT('Origin',(-4.44089209850063E-17,-0.02400000000001,
6.72997231505748E-33));
#33553=CARTESIAN_POINT('',(-0.00433948917003908,-0.024,0.0122543393841983));
#33554=CARTESIAN_POINT('',(-0.00433948917004908,-0.02400000000001,0.0122543393842083));
#33555=CARTESIAN_POINT('Origin',(-4.44089209850063E-17,-0.02400000000001,
6.72997231505748E-33));
#33556=CARTESIAN_POINT('Origin',(-4.44089209850063E-17,-0.02400000000001,
6.72997231505748E-33));
#33557=CARTESIAN_POINT('',(-0.00043494423791826,-0.024,0.0129927219438385));
#33558=CARTESIAN_POINT('Origin',(-4.44089209850063E-17,-0.02400000000001,
6.72997231505748E-33));
#33559=CARTESIAN_POINT('',(-0.000443640587169973,-0.02400000000001,0.0132525006413773));
#33560=CARTESIAN_POINT('Origin',(-4.44089209850063E-17,-0.02400000000001,
6.72997231505748E-33));
#33561=CARTESIAN_POINT('Origin',(-4.44089209850063E-17,-0.016,6.72997231505748E-33));
#33562=CARTESIAN_POINT('',(-0.00043494423791826,-0.008,0.0129927219438385));
#33563=CARTESIAN_POINT('Origin',(-4.44089209850063E-17,-0.00799999999999,
6.72997231505748E-33));
#33564=CARTESIAN_POINT('',(-0.000434944237928261,-0.016,0.0129927219438485));
#33565=CARTESIAN_POINT('Origin',(-4.44089209850063E-17,-0.016,6.72997231505748E-33));
#33566=CARTESIAN_POINT('',(-0.00433948917003908,-0.008,0.0122543393841983));
#33567=CARTESIAN_POINT('',(-0.00433948917004908,-0.016,0.0122543393842083));
#33568=CARTESIAN_POINT('Origin',(-4.44089209850063E-17,-0.00799999999999,
6.72997231505748E-33));
#33569=CARTESIAN_POINT('Origin',(-0.000450000000000044,-0.008,0.0134424700111252));
#33570=CARTESIAN_POINT('',(-0.000443640587169973,-0.00799999999999,0.0132525006413773));
#33571=CARTESIAN_POINT('Origin',(-4.44089209850063E-17,-0.016,6.72997231505748E-33));
#33572=CARTESIAN_POINT('Origin',(-4.44089209850063E-17,-0.00799999999999,
6.72997231505748E-33));
#33573=CARTESIAN_POINT('Origin',(-4.44089209850063E-17,-0.016,6.72997231505748E-33));
#33574=CARTESIAN_POINT('',(0.00463991534334938,-0.008,0.0131027167261813));
#33575=CARTESIAN_POINT('',(0.00463991534335938,-0.016,0.0131027167261913));
#33576=CARTESIAN_POINT('',(-0.00463991534334946,-0.008,0.0131027167261813));
#33577=CARTESIAN_POINT('Origin',(-4.44089209850063E-17,-0.00799999999999,
6.72997231505748E-33));
#33578=CARTESIAN_POINT('',(-0.00463991534335947,-0.016,0.0131027167261913));
#33579=CARTESIAN_POINT('Origin',(-0.00433948917003908,-0.016,0.0122543393841983));
#33580=CARTESIAN_POINT('',(-0.00433948917004908,-0.00799999999999,0.0122543393842083));
#33581=CARTESIAN_POINT('Origin',(-4.44089209850063E-17,-0.016,6.72997231505748E-33));
#33582=CARTESIAN_POINT('Origin',(-4.44089209850063E-17,-0.00799999999999,
6.72997231505748E-33));
#33583=CARTESIAN_POINT('Origin',(0.00463991534334938,-0.016,0.0131027167261813));
#33584=CARTESIAN_POINT('',(0.00463991534335938,-0.00799999999999,0.0131027167261913));
#33585=CARTESIAN_POINT('Origin',(-4.57966997657877E-17,-0.008,0.0130771696920992));
#34833=UNCERTAINTY_MEASURE_WITH_UNIT(LENGTH_MEASURE(1.E-5),#34877,
'DISTANCE_ACCURACY_VALUE',
'Maximum model space distance between geometric entities at asserted c
onnectivities');
#34841=UNCERTAINTY_MEASURE_WITH_UNIT(LENGTH_MEASURE(1.E-5),#34877,
'DISTANCE_ACCURACY_VALUE',
'Maximum model space distance between geometric entities at asserted c
onnectivities');
#34868=(
GEOMETRIC_REPRESENTATION_CONTEXT(3)
GLOBAL_UNCERTAINTY_ASSIGNED_CONTEXT((#34833))
GLOBAL_UNIT_ASSIGNED_CONTEXT((#34877,#34878,#34879))
REPRESENTATION_CONTEXT('','3D')
);
#34876=(
GEOMETRIC_REPRESENTATION_CONTEXT(3)
GLOBAL_UNCERTAINTY_ASSIGNED_CONTEXT((#34841))
GLOBAL_UNIT_ASSIGNED_CONTEXT((#34877,#34878,#34879))
REPRESENTATION_CONTEXT('','3D')
);
#34877=(
LENGTH_UNIT()
NAMED_UNIT(*)
SI_UNIT($,.METRE.)
);
#34878=(
NAMED_UNIT(*)
PLANE_ANGLE_UNIT()
SI_UNIT($,.RADIAN.)
);
#34879=(
NAMED_UNIT(*)
SI_UNIT($,.STERADIAN.)
SOLID_ANGLE_UNIT()
);
#34906=SHAPE_DEFINITION_REPRESENTATION(#34940,#35010);
#34940=PRODUCT_DEFINITION_SHAPE('',$,#35045);
#35010=SHAPE_REPRESENTATION('',(#21823),#34868);
#35018=PRODUCT_DEFINITION_CONTEXT('part definition',#35122,'design');
#35045=PRODUCT_DEFINITION('Motor Stator Face 6','Motor Stator Face 6',#35079,
#35018);
#35079=PRODUCT_DEFINITION_FORMATION('',$,#35150);
#35122=APPLICATION_CONTEXT('Managed model based 3d engineering');
#35123=PRODUCT_CONTEXT('part definition',#35122,'mechanical');
#35150=PRODUCT('Motor Stator Face 6','Motor Stator Face 6',
'LEGAL AND USAGE DISCLAIMER: this Data/Model is provided \X2\201C\X0\A
S IS\X2\201D\X0\ for informational and representational only. It is a 
geometric approximation and is NOT engineered, certified, or guarantee
d for dimensional accuracy, exact tolerances, or production-level prec
ision. Vendor disclaims all implied warranties including fitness for a
 particular purpose. DO NOT USE FOR DIRECT PHYSICAL MANUFACTURING, AUT
OMATED PRODUCTION, OR SAFETY-CRITICAL SYSTEMS without independent engi
neering verification and resolution of any design discrepancies.',(#35123));
#35160=PRESENTATION_STYLE_ASSIGNMENT((#35169));
#35169=SURFACE_STYLE_USAGE(.BOTH.,#35178);
#35178=SURFACE_SIDE_STYLE('',(#35187));
#35187=SURFACE_STYLE_FILL_AREA(#35196);
#35196=FILL_AREA_STYLE('Plastic - Glossy (Black)',(#35205));
#35205=FILL_AREA_STYLE_COLOUR('Plastic - Glossy (Black)',#35214);
#35214=COLOUR_RGB('Plastic - Glossy (Black)',0.0980392156862745,0.0980392156862745,
0.0980392156862745);
ENDSEC;
END-ISO-10303-21;
